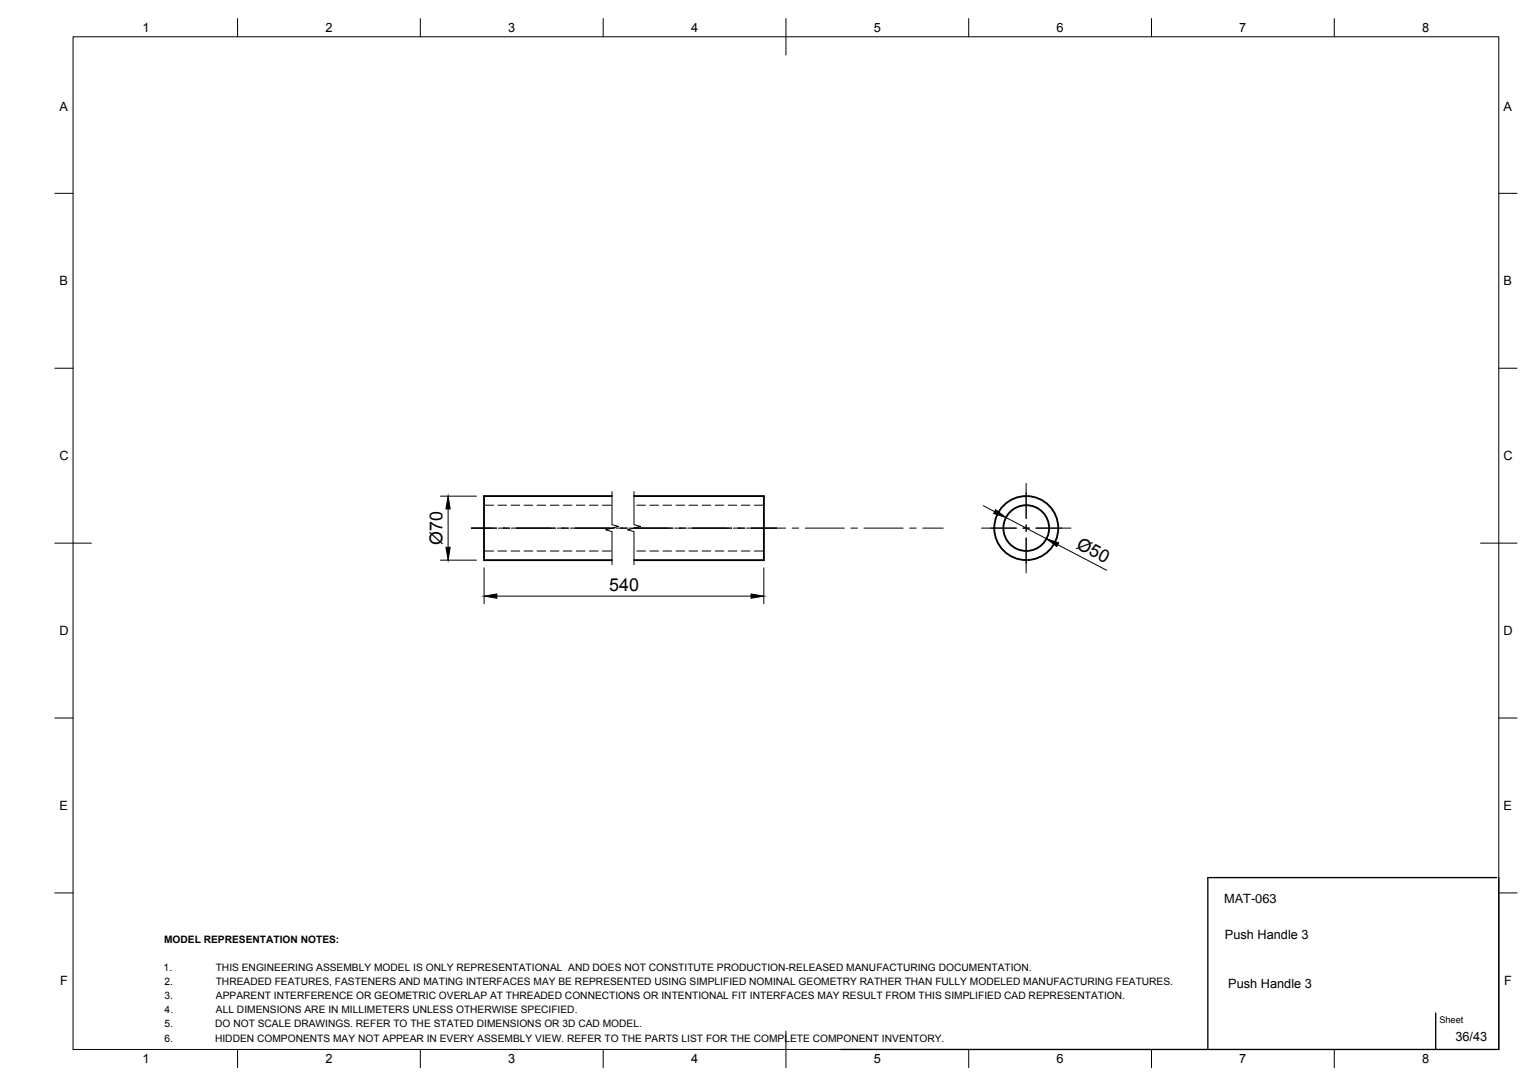
ISO-10303-21;
HEADER;
/* Generated by software containing ST-Developer
 * from STEP Tools, Inc. (www.steptools.com) 
 */

FILE_DESCRIPTION(
/* description */ (''),
/* implementation_level */ '2;1');

FILE_NAME(
/* name */ 'Push Handle 3.step',
/* time_stamp */ '2026-10-24T09:43:01-07:00',
/* author */ (''),
/* organization */ (''),
/* preprocessor_version */ 'ST-DEVELOPER v20.2',
/* originating_system */ 'Autodesk Translation Framework v15.15.0.0',
/* authorisation */ '');

FILE_SCHEMA (('AUTOMOTIVE_DESIGN { 1 0 10303 214 3 1 1 }'));
ENDSEC;

DATA;
#10=MECHANICAL_DESIGN_GEOMETRIC_PRESENTATION_REPRESENTATION('',(#299),#11112);
#233=SHAPE_REPRESENTATION_RELATIONSHIP('SRR','None',#11259,#266);
#266=ADVANCED_BREP_SHAPE_REPRESENTATION('',(#332),#11104);
#299=STYLED_ITEM('',(#11426),#332);
#332=MANIFOLD_SOLID_BREP('Push Handle 3',#6036);
#479=FACE_BOUND('',#1509,.T.);
#480=FACE_BOUND('',#1511,.T.);
#650=PLANE('',#7162);
#651=PLANE('',#7164);
#1003=FACE_OUTER_BOUND('',#1507,.T.);
#1004=FACE_OUTER_BOUND('',#1508,.T.);
#1005=FACE_OUTER_BOUND('',#1510,.T.);
#1006=FACE_OUTER_BOUND('',#1512,.T.);
#1507=EDGE_LOOP('',(#5381,#5382,#5383,#5384));
#1508=EDGE_LOOP('',(#5385));
#1509=EDGE_LOOP('',(#5386));
#1510=EDGE_LOOP('',(#5387));
#1511=EDGE_LOOP('',(#5388));
#1512=EDGE_LOOP('',(#5389,#5390,#5391,#5392));
#1894=LINE('',#10875,#2253);
#1895=LINE('',#10884,#2254);
#2253=VECTOR('',#9104,0.025);
#2254=VECTOR('',#9117,0.035);
#2650=CIRCLE('',#7160,0.025);
#2651=CIRCLE('',#7161,0.025);
#2652=CIRCLE('',#7163,0.035);
#2653=CIRCLE('',#7165,0.035);
#3140=VERTEX_POINT('',#10872);
#3141=VERTEX_POINT('',#10874);
#3142=VERTEX_POINT('',#10878);
#3143=VERTEX_POINT('',#10881);
#3894=EDGE_CURVE('',#3140,#3140,#2650,.T.);
#3895=EDGE_CURVE('',#3140,#3141,#1894,.T.);
#3896=EDGE_CURVE('',#3141,#3141,#2651,.F.);
#3897=EDGE_CURVE('',#3142,#3142,#2652,.F.);
#3898=EDGE_CURVE('',#3143,#3143,#2653,.F.);
#3899=EDGE_CURVE('',#3142,#3143,#1895,.T.);
#5381=ORIENTED_EDGE('',*,*,#3894,.F.);
#5382=ORIENTED_EDGE('',*,*,#3895,.T.);
#5383=ORIENTED_EDGE('',*,*,#3896,.F.);
#5384=ORIENTED_EDGE('',*,*,#3895,.F.);
#5385=ORIENTED_EDGE('',*,*,#3897,.F.);
#5386=ORIENTED_EDGE('',*,*,#3896,.T.);
#5387=ORIENTED_EDGE('',*,*,#3898,.T.);
#5388=ORIENTED_EDGE('',*,*,#3894,.T.);
#5389=ORIENTED_EDGE('',*,*,#3897,.T.);
#5390=ORIENTED_EDGE('',*,*,#3899,.T.);
#5391=ORIENTED_EDGE('',*,*,#3898,.F.);
#5392=ORIENTED_EDGE('',*,*,#3899,.F.);
#5627=CYLINDRICAL_SURFACE('',#7159,0.025);
#5628=CYLINDRICAL_SURFACE('',#7166,0.035);
#5976=ADVANCED_FACE('',(#1003),#5627,.F.);
#5977=ADVANCED_FACE('',(#1004,#479),#650,.F.);
#5978=ADVANCED_FACE('',(#1005,#480),#651,.T.);
#5979=ADVANCED_FACE('',(#1006),#5628,.T.);
#6036=CLOSED_SHELL('',(#5976,#5977,#5978,#5979));
#7158=AXIS2_PLACEMENT_3D('',#10870,#9098,#9099);
#7159=AXIS2_PLACEMENT_3D('',#10871,#9100,#9101);
#7160=AXIS2_PLACEMENT_3D('',#10873,#9102,#9103);
#7161=AXIS2_PLACEMENT_3D('',#10876,#9105,#9106);
#7162=AXIS2_PLACEMENT_3D('',#10877,#9107,#9108);
#7163=AXIS2_PLACEMENT_3D('',#10879,#9109,#9110);
#7164=AXIS2_PLACEMENT_3D('',#10880,#9111,#9112);
#7165=AXIS2_PLACEMENT_3D('',#10882,#9113,#9114);
#7166=AXIS2_PLACEMENT_3D('',#10883,#9115,#9116);
#9098=DIRECTION('axis',(0.,0.,1.));
#9099=DIRECTION('refdir',(1.,0.,0.));
#9100=DIRECTION('center_axis',(-1.,0.,0.));
#9101=DIRECTION('ref_axis',(0.,0.,1.));
#9102=DIRECTION('center_axis',(-1.,0.,0.));
#9103=DIRECTION('ref_axis',(0.,0.,1.));
#9104=DIRECTION('',(-1.,0.,0.));
#9105=DIRECTION('center_axis',(-1.,0.,0.));
#9106=DIRECTION('ref_axis',(0.,0.,1.));
#9107=DIRECTION('center_axis',(1.,0.,0.));
#9108=DIRECTION('ref_axis',(0.,0.,-1.));
#9109=DIRECTION('center_axis',(-1.,0.,0.));
#9110=DIRECTION('ref_axis',(0.,0.,1.));
#9111=DIRECTION('center_axis',(1.,0.,0.));
#9112=DIRECTION('ref_axis',(0.,0.,-1.));
#9113=DIRECTION('center_axis',(-1.,0.,0.));
#9114=DIRECTION('ref_axis',(0.,0.,1.));
#9115=DIRECTION('center_axis',(-1.,0.,0.));
#9116=DIRECTION('ref_axis',(0.,0.,1.));
#9117=DIRECTION('',(1.,0.,0.));
#10870=CARTESIAN_POINT('',(0.,0.,0.));
#10871=CARTESIAN_POINT('Origin',(0.27,0.69,-1.3));
#10872=CARTESIAN_POINT('',(0.27,0.69,-1.325));
#10873=CARTESIAN_POINT('Origin',(0.27,0.69,-1.3));
#10874=CARTESIAN_POINT('',(-0.27,0.69,-1.325));
#10875=CARTESIAN_POINT('',(0.27,0.69,-1.325));
#10876=CARTESIAN_POINT('Origin',(-0.27,0.69,-1.3));
#10877=CARTESIAN_POINT('Origin',(-0.27,0.69,-1.3));
#10878=CARTESIAN_POINT('',(-0.27,0.69,-1.335));
#10879=CARTESIAN_POINT('Origin',(-0.27,0.69,-1.3));
#10880=CARTESIAN_POINT('Origin',(0.27,0.69,-1.3));
#10881=CARTESIAN_POINT('',(0.27,0.69,-1.335));
#10882=CARTESIAN_POINT('Origin',(0.27,0.69,-1.3));
#10883=CARTESIAN_POINT('Origin',(0.27,0.69,-1.3));
#10884=CARTESIAN_POINT('',(0.27,0.69,-1.335));
#11065=UNCERTAINTY_MEASURE_WITH_UNIT(LENGTH_MEASURE(1.E-5),#11113,
'DISTANCE_ACCURACY_VALUE',
'Maximum model space distance between geometric entities at asserted c
onnectivities');
#11073=UNCERTAINTY_MEASURE_WITH_UNIT(LENGTH_MEASURE(1.E-5),#11113,
'DISTANCE_ACCURACY_VALUE',
'Maximum model space distance between geometric entities at asserted c
onnectivities');
#11104=(
GEOMETRIC_REPRESENTATION_CONTEXT(3)
GLOBAL_UNCERTAINTY_ASSIGNED_CONTEXT((#11065))
GLOBAL_UNIT_ASSIGNED_CONTEXT((#11113,#11114,#11115))
REPRESENTATION_CONTEXT('','3D')
);
#11112=(
GEOMETRIC_REPRESENTATION_CONTEXT(3)
GLOBAL_UNCERTAINTY_ASSIGNED_CONTEXT((#11073))
GLOBAL_UNIT_ASSIGNED_CONTEXT((#11113,#11114,#11115))
REPRESENTATION_CONTEXT('','3D')
);
#11113=(
LENGTH_UNIT()
NAMED_UNIT(*)
SI_UNIT($,.METRE.)
);
#11114=(
NAMED_UNIT(*)
PLANE_ANGLE_UNIT()
SI_UNIT($,.RADIAN.)
);
#11115=(
NAMED_UNIT(*)
SI_UNIT($,.STERADIAN.)
SOLID_ANGLE_UNIT()
);
#11146=SHAPE_DEFINITION_REPRESENTATION(#11197,#11259);
#11197=PRODUCT_DEFINITION_SHAPE('',$,#11298);
#11259=SHAPE_REPRESENTATION('',(#7158),#11104);
#11267=PRODUCT_DEFINITION_CONTEXT('part definition',#11383,'design');
#11298=PRODUCT_DEFINITION('Push Handle 3','Push Handle 3',#11336,#11267);
#11336=PRODUCT_DEFINITION_FORMATION('',$,#11415);
#11383=APPLICATION_CONTEXT(
'Core Data for Automotive Mechanical Design Process');
#11384=PRODUCT_CONTEXT('part definition',#11383,'mechanical');
#11415=PRODUCT('Push Handle 3','Push Handle 3',
'back_push__ DE     3061',(#11384));
#11426=PRESENTATION_STYLE_ASSIGNMENT((#11430));
#11430=SURFACE_STYLE_USAGE(.BOTH.,#11434);
#11434=SURFACE_SIDE_STYLE('',(#11438));
#11438=SURFACE_STYLE_FILL_AREA(#11442);
#11442=FILL_AREA_STYLE('Opaque(202,209,238)',(#11446));
#11446=FILL_AREA_STYLE_COLOUR('Opaque(202,209,238)',#11450);
#11450=COLOUR_RGB('Opaque(202,209,238)',0.792156862745098,0.819607843137255,
0.933333333333333);
ENDSEC;
END-ISO-10303-21;
